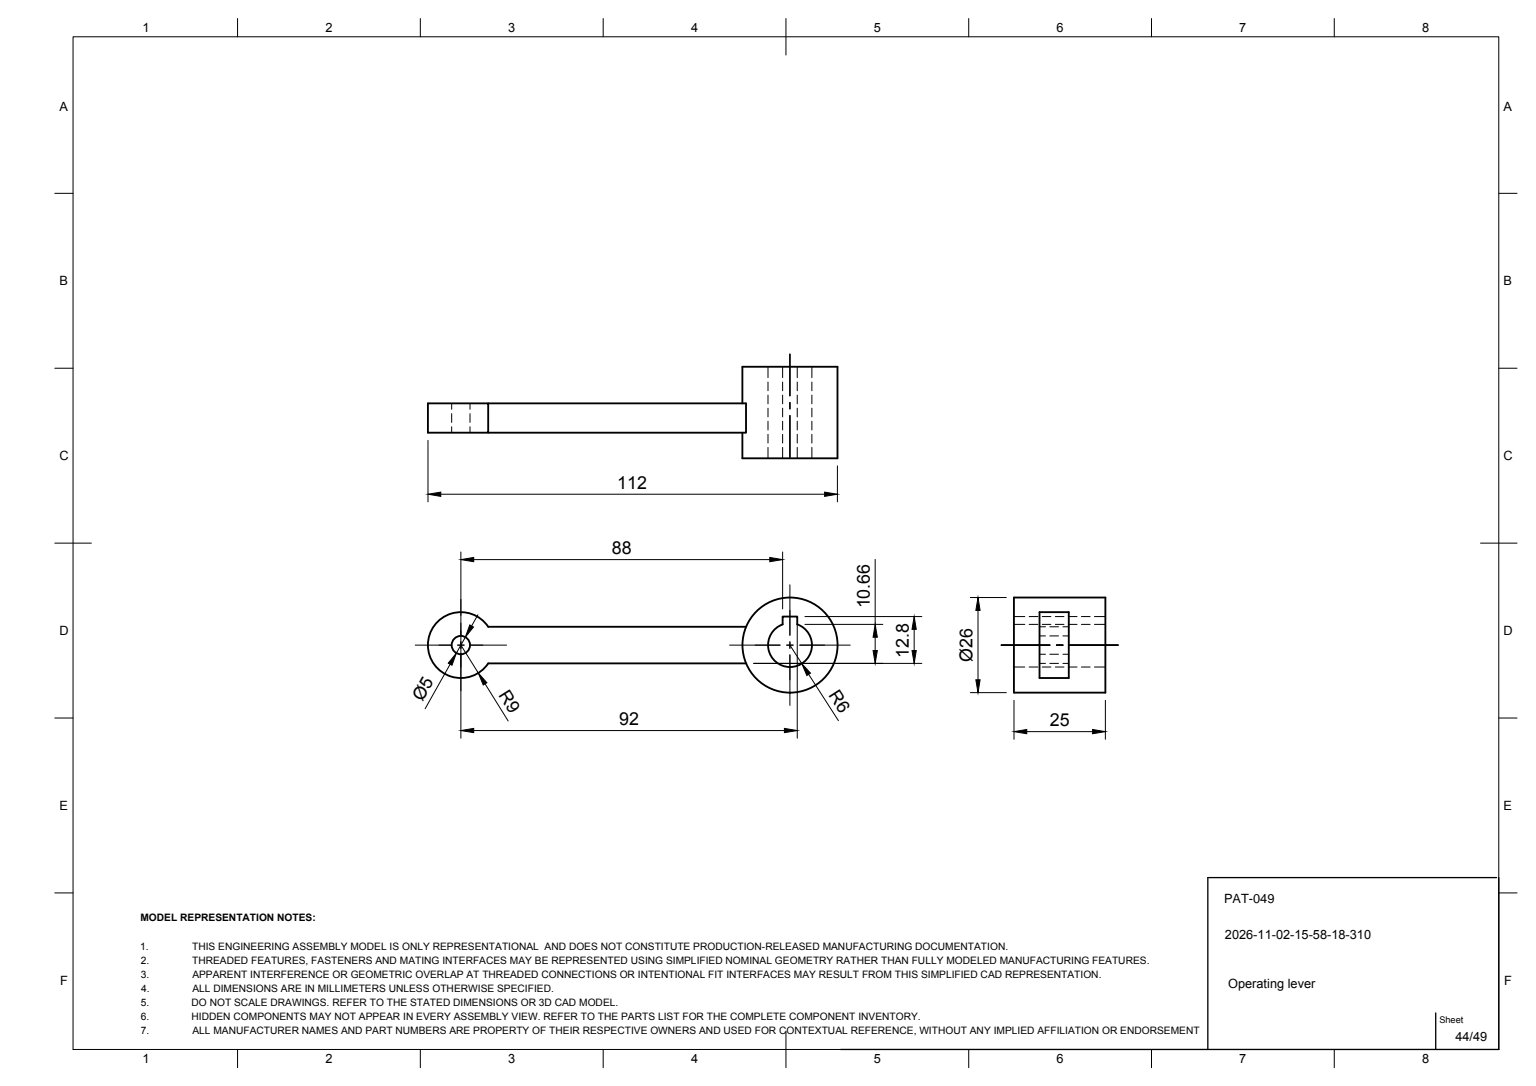
ISO-10303-21;
HEADER;
/* Generated by software containing ST-Developer
 * from STEP Tools, Inc. (www.steptools.com) 
 */

FILE_DESCRIPTION(
/* description */ ('Hand drill press frame (manual)'),
/* implementation_level */ '2;1');

FILE_NAME(
/* name */ 'Operating lever.step',
/* time_stamp */ '2026-10-28T03:25:28-07:00',
/* author */ (''),
/* organization */ (''),
/* preprocessor_version */ 'ST-DEVELOPER v20.2',
/* originating_system */ 'Autodesk Translation Framework v15.17.0.0',
/* authorisation */ '');

FILE_SCHEMA (('AUTOMOTIVE_DESIGN { 1 0 10303 214 3 1 1 }'));
ENDSEC;

DATA;
#10=MECHANICAL_DESIGN_GEOMETRIC_PRESENTATION_REPRESENTATION('',(#662),#33299);
#565=SHAPE_REPRESENTATION_RELATIONSHIP('SRR','None',#33527,#610);
#610=ADVANCED_BREP_SHAPE_REPRESENTATION('',(#713),#33289);
#662=STYLED_ITEM('',(#33800),#713);
#713=MANIFOLD_SOLID_BREP('Body1',#12681);
#867=FACE_BOUND('',#2714,.T.);
#868=FACE_BOUND('',#2719,.T.);
#869=FACE_BOUND('',#2722,.T.);
#870=FACE_BOUND('',#2724,.T.);
#871=FACE_BOUND('',#2726,.T.);
#1272=PLANE('',#14087);
#1273=PLANE('',#14088);
#1274=PLANE('',#14089);
#1275=PLANE('',#14090);
#1276=PLANE('',#14098);
#1277=PLANE('',#14099);
#1278=PLANE('',#14101);
#1279=PLANE('',#14102);
#1280=PLANE('',#14106);
#1873=FACE_OUTER_BOUND('',#2709,.T.);
#1874=FACE_OUTER_BOUND('',#2710,.T.);
#1875=FACE_OUTER_BOUND('',#2711,.T.);
#1876=FACE_OUTER_BOUND('',#2712,.T.);
#1877=FACE_OUTER_BOUND('',#2713,.T.);
#1878=FACE_OUTER_BOUND('',#2715,.T.);
#1879=FACE_OUTER_BOUND('',#2716,.T.);
#1880=FACE_OUTER_BOUND('',#2717,.T.);
#1881=FACE_OUTER_BOUND('',#2718,.T.);
#1882=FACE_OUTER_BOUND('',#2720,.T.);
#1883=FACE_OUTER_BOUND('',#2721,.T.);
#1884=FACE_OUTER_BOUND('',#2723,.T.);
#1885=FACE_OUTER_BOUND('',#2725,.T.);
#2709=EDGE_LOOP('',(#11027,#11028,#11029,#11030));
#2710=EDGE_LOOP('',(#11031,#11032,#11033,#11034));
#2711=EDGE_LOOP('',(#11035,#11036,#11037,#11038));
#2712=EDGE_LOOP('',(#11039,#11040,#11041,#11042));
#2713=EDGE_LOOP('',(#11043));
#2714=EDGE_LOOP('',(#11044,#11045,#11046,#11047));
#2715=EDGE_LOOP('',(#11048,#11049,#11050,#11051));
#2716=EDGE_LOOP('',(#11052,#11053,#11054,#11055));
#2717=EDGE_LOOP('',(#11056,#11057,#11058,#11059));
#2718=EDGE_LOOP('',(#11060,#11061,#11062,#11063));
#2719=EDGE_LOOP('',(#11064));
#2720=EDGE_LOOP('',(#11065,#11066,#11067,#11068));
#2721=EDGE_LOOP('',(#11069,#11070,#11071,#11072));
#2722=EDGE_LOOP('',(#11073));
#2723=EDGE_LOOP('',(#11074,#11075,#11076,#11077));
#2724=EDGE_LOOP('',(#11078,#11079,#11080,#11081));
#2725=EDGE_LOOP('',(#11082));
#2726=EDGE_LOOP('',(#11083,#11084,#11085,#11086));
#3840=LINE('',#21258,#5005);
#3841=LINE('',#21263,#5006);
#3842=LINE('',#21265,#5007);
#3843=LINE('',#21267,#5008);
#3844=LINE('',#21268,#5009);
#3845=LINE('',#21271,#5010);
#3846=LINE('',#21273,#5011);
#3847=LINE('',#21274,#5012);
#3848=LINE('',#21277,#5013);
#3849=LINE('',#21279,#5014);
#3850=LINE('',#21280,#5015);
#3851=LINE('',#21290,#5016);
#3852=LINE('',#21294,#5017);
#3853=LINE('',#21298,#5018);
#3854=LINE('',#21300,#5019);
#3855=LINE('',#21301,#5020);
#3856=LINE('',#21304,#5021);
#3857=LINE('',#21308,#5022);
#3858=LINE('',#21309,#5023);
#3859=LINE('',#21314,#5024);
#5005=VECTOR('',#17119,0.25);
#5006=VECTOR('',#17124,1.);
#5007=VECTOR('',#17125,1.);
#5008=VECTOR('',#17126,1.);
#5009=VECTOR('',#17127,1.);
#5010=VECTOR('',#17130,1.);
#5011=VECTOR('',#17131,1.);
#5012=VECTOR('',#17132,1.);
#5013=VECTOR('',#17135,1.);
#5014=VECTOR('',#17136,1.);
#5015=VECTOR('',#17137,1.);
#5016=VECTOR('',#17150,1.);
#5017=VECTOR('',#17153,1.);
#5018=VECTOR('',#17158,1.);
#5019=VECTOR('',#17159,1.);
#5020=VECTOR('',#17160,1.);
#5021=VECTOR('',#17163,1.);
#5022=VECTOR('',#17168,1.);
#5023=VECTOR('',#17169,1.);
#5024=VECTOR('',#17176,1.3);
#5523=CIRCLE('',#14085,0.25);
#5524=CIRCLE('',#14086,0.25);
#5525=CIRCLE('',#14091,1.3);
#5526=CIRCLE('',#14092,0.6);
#5527=CIRCLE('',#14094,0.6);
#5528=CIRCLE('',#14096,0.9);
#5529=CIRCLE('',#14097,0.9);
#5530=CIRCLE('',#14100,1.3);
#5531=CIRCLE('',#14103,1.3);
#5532=CIRCLE('',#14105,1.3);
#6489=VERTEX_POINT('',#21255);
#6490=VERTEX_POINT('',#21257);
#6491=VERTEX_POINT('',#21261);
#6492=VERTEX_POINT('',#21262);
#6493=VERTEX_POINT('',#21264);
#6494=VERTEX_POINT('',#21266);
#6495=VERTEX_POINT('',#21270);
#6496=VERTEX_POINT('',#21272);
#6497=VERTEX_POINT('',#21276);
#6498=VERTEX_POINT('',#21278);
#6499=VERTEX_POINT('',#21282);
#6500=VERTEX_POINT('',#21288);
#6501=VERTEX_POINT('',#21289);
#6502=VERTEX_POINT('',#21291);
#6503=VERTEX_POINT('',#21293);
#6504=VERTEX_POINT('',#21297);
#6505=VERTEX_POINT('',#21299);
#6506=VERTEX_POINT('',#21303);
#6507=VERTEX_POINT('',#21307);
#6508=VERTEX_POINT('',#21313);
#8042=EDGE_CURVE('',#6489,#6489,#5523,.T.);
#8043=EDGE_CURVE('',#6489,#6490,#3840,.T.);
#8044=EDGE_CURVE('',#6490,#6490,#5524,.T.);
#8045=EDGE_CURVE('',#6491,#6492,#3841,.T.);
#8046=EDGE_CURVE('',#6491,#6493,#3842,.T.);
#8047=EDGE_CURVE('',#6494,#6493,#3843,.T.);
#8048=EDGE_CURVE('',#6492,#6494,#3844,.T.);
#8049=EDGE_CURVE('',#6495,#6491,#3845,.T.);
#8050=EDGE_CURVE('',#6495,#6496,#3846,.T.);
#8051=EDGE_CURVE('',#6493,#6496,#3847,.T.);
#8052=EDGE_CURVE('',#6497,#6495,#3848,.T.);
#8053=EDGE_CURVE('',#6498,#6497,#3849,.T.);
#8054=EDGE_CURVE('',#6496,#6498,#3850,.T.);
#8055=EDGE_CURVE('',#6499,#6499,#5525,.T.);
#8056=EDGE_CURVE('',#6498,#6494,#5526,.T.);
#8057=EDGE_CURVE('',#6497,#6492,#5527,.T.);
#8058=EDGE_CURVE('',#6500,#6501,#3851,.T.);
#8059=EDGE_CURVE('',#6502,#6500,#5528,.T.);
#8060=EDGE_CURVE('',#6503,#6502,#3852,.T.);
#8061=EDGE_CURVE('',#6503,#6501,#5529,.T.);
#8062=EDGE_CURVE('',#6504,#6501,#3853,.T.);
#8063=EDGE_CURVE('',#6505,#6504,#3854,.T.);
#8064=EDGE_CURVE('',#6500,#6505,#3855,.T.);
#8065=EDGE_CURVE('',#6503,#6506,#3856,.T.);
#8066=EDGE_CURVE('',#6504,#6506,#5530,.T.);
#8067=EDGE_CURVE('',#6507,#6502,#3857,.T.);
#8068=EDGE_CURVE('',#6506,#6507,#3858,.T.);
#8069=EDGE_CURVE('',#6507,#6505,#5531,.T.);
#8070=EDGE_CURVE('',#6499,#6508,#3859,.T.);
#8071=EDGE_CURVE('',#6508,#6508,#5532,.T.);
#11027=ORIENTED_EDGE('',*,*,#8042,.F.);
#11028=ORIENTED_EDGE('',*,*,#8043,.T.);
#11029=ORIENTED_EDGE('',*,*,#8044,.F.);
#11030=ORIENTED_EDGE('',*,*,#8043,.F.);
#11031=ORIENTED_EDGE('',*,*,#8045,.F.);
#11032=ORIENTED_EDGE('',*,*,#8046,.T.);
#11033=ORIENTED_EDGE('',*,*,#8047,.F.);
#11034=ORIENTED_EDGE('',*,*,#8048,.F.);
#11035=ORIENTED_EDGE('',*,*,#8049,.F.);
#11036=ORIENTED_EDGE('',*,*,#8050,.T.);
#11037=ORIENTED_EDGE('',*,*,#8051,.F.);
#11038=ORIENTED_EDGE('',*,*,#8046,.F.);
#11039=ORIENTED_EDGE('',*,*,#8052,.F.);
#11040=ORIENTED_EDGE('',*,*,#8053,.F.);
#11041=ORIENTED_EDGE('',*,*,#8054,.F.);
#11042=ORIENTED_EDGE('',*,*,#8050,.F.);
#11043=ORIENTED_EDGE('',*,*,#8055,.T.);
#11044=ORIENTED_EDGE('',*,*,#8047,.T.);
#11045=ORIENTED_EDGE('',*,*,#8051,.T.);
#11046=ORIENTED_EDGE('',*,*,#8054,.T.);
#11047=ORIENTED_EDGE('',*,*,#8056,.T.);
#11048=ORIENTED_EDGE('',*,*,#8048,.T.);
#11049=ORIENTED_EDGE('',*,*,#8056,.F.);
#11050=ORIENTED_EDGE('',*,*,#8053,.T.);
#11051=ORIENTED_EDGE('',*,*,#8057,.T.);
#11052=ORIENTED_EDGE('',*,*,#8058,.F.);
#11053=ORIENTED_EDGE('',*,*,#8059,.F.);
#11054=ORIENTED_EDGE('',*,*,#8060,.F.);
#11055=ORIENTED_EDGE('',*,*,#8061,.T.);
#11056=ORIENTED_EDGE('',*,*,#8058,.T.);
#11057=ORIENTED_EDGE('',*,*,#8062,.F.);
#11058=ORIENTED_EDGE('',*,*,#8063,.F.);
#11059=ORIENTED_EDGE('',*,*,#8064,.F.);
#11060=ORIENTED_EDGE('',*,*,#8061,.F.);
#11061=ORIENTED_EDGE('',*,*,#8065,.T.);
#11062=ORIENTED_EDGE('',*,*,#8066,.F.);
#11063=ORIENTED_EDGE('',*,*,#8062,.T.);
#11064=ORIENTED_EDGE('',*,*,#8042,.T.);
#11065=ORIENTED_EDGE('',*,*,#8060,.T.);
#11066=ORIENTED_EDGE('',*,*,#8067,.F.);
#11067=ORIENTED_EDGE('',*,*,#8068,.F.);
#11068=ORIENTED_EDGE('',*,*,#8065,.F.);
#11069=ORIENTED_EDGE('',*,*,#8064,.T.);
#11070=ORIENTED_EDGE('',*,*,#8069,.F.);
#11071=ORIENTED_EDGE('',*,*,#8067,.T.);
#11072=ORIENTED_EDGE('',*,*,#8059,.T.);
#11073=ORIENTED_EDGE('',*,*,#8044,.T.);
#11074=ORIENTED_EDGE('',*,*,#8055,.F.);
#11075=ORIENTED_EDGE('',*,*,#8070,.T.);
#11076=ORIENTED_EDGE('',*,*,#8071,.T.);
#11077=ORIENTED_EDGE('',*,*,#8070,.F.);
#11078=ORIENTED_EDGE('',*,*,#8063,.T.);
#11079=ORIENTED_EDGE('',*,*,#8066,.T.);
#11080=ORIENTED_EDGE('',*,*,#8068,.T.);
#11081=ORIENTED_EDGE('',*,*,#8069,.T.);
#11082=ORIENTED_EDGE('',*,*,#8071,.F.);
#11083=ORIENTED_EDGE('',*,*,#8045,.T.);
#11084=ORIENTED_EDGE('',*,*,#8057,.F.);
#11085=ORIENTED_EDGE('',*,*,#8052,.T.);
#11086=ORIENTED_EDGE('',*,*,#8049,.T.);
#11908=CYLINDRICAL_SURFACE('',#14084,0.25);
#11909=CYLINDRICAL_SURFACE('',#14093,0.6);
#11910=CYLINDRICAL_SURFACE('',#14095,0.9);
#11911=CYLINDRICAL_SURFACE('',#14104,1.3);
#12482=ADVANCED_FACE('',(#1873),#11908,.F.);
#12483=ADVANCED_FACE('',(#1874),#1272,.F.);
#12484=ADVANCED_FACE('',(#1875),#1273,.F.);
#12485=ADVANCED_FACE('',(#1876),#1274,.F.);
#12486=ADVANCED_FACE('',(#1877,#867),#1275,.T.);
#12487=ADVANCED_FACE('',(#1878),#11909,.F.);
#12488=ADVANCED_FACE('',(#1879),#11910,.T.);
#12489=ADVANCED_FACE('',(#1880),#1276,.T.);
#12490=ADVANCED_FACE('',(#1881,#868),#1277,.F.);
#12491=ADVANCED_FACE('',(#1882),#1278,.T.);
#12492=ADVANCED_FACE('',(#1883,#869),#1279,.T.);
#12493=ADVANCED_FACE('',(#1884,#870),#11911,.T.);
#12494=ADVANCED_FACE('',(#1885,#871),#1280,.F.);
#12681=CLOSED_SHELL('',(#12482,#12483,#12484,#12485,#12486,#12487,#12488,
#12489,#12490,#12491,#12492,#12493,#12494));
#14083=AXIS2_PLACEMENT_3D('',#21253,#17113,#17114);
#14084=AXIS2_PLACEMENT_3D('',#21254,#17115,#17116);
#14085=AXIS2_PLACEMENT_3D('',#21256,#17117,#17118);
#14086=AXIS2_PLACEMENT_3D('',#21259,#17120,#17121);
#14087=AXIS2_PLACEMENT_3D('',#21260,#17122,#17123);
#14088=AXIS2_PLACEMENT_3D('',#21269,#17128,#17129);
#14089=AXIS2_PLACEMENT_3D('',#21275,#17133,#17134);
#14090=AXIS2_PLACEMENT_3D('',#21281,#17138,#17139);
#14091=AXIS2_PLACEMENT_3D('',#21283,#17140,#17141);
#14092=AXIS2_PLACEMENT_3D('',#21284,#17142,#17143);
#14093=AXIS2_PLACEMENT_3D('',#21285,#17144,#17145);
#14094=AXIS2_PLACEMENT_3D('',#21286,#17146,#17147);
#14095=AXIS2_PLACEMENT_3D('',#21287,#17148,#17149);
#14096=AXIS2_PLACEMENT_3D('',#21292,#17151,#17152);
#14097=AXIS2_PLACEMENT_3D('',#21295,#17154,#17155);
#14098=AXIS2_PLACEMENT_3D('',#21296,#17156,#17157);
#14099=AXIS2_PLACEMENT_3D('',#21302,#17161,#17162);
#14100=AXIS2_PLACEMENT_3D('',#21305,#17164,#17165);
#14101=AXIS2_PLACEMENT_3D('',#21306,#17166,#17167);
#14102=AXIS2_PLACEMENT_3D('',#21310,#17170,#17171);
#14103=AXIS2_PLACEMENT_3D('',#21311,#17172,#17173);
#14104=AXIS2_PLACEMENT_3D('',#21312,#17174,#17175);
#14105=AXIS2_PLACEMENT_3D('',#21315,#17177,#17178);
#14106=AXIS2_PLACEMENT_3D('',#21316,#17179,#17180);
#17113=DIRECTION('axis',(0.,0.,1.));
#17114=DIRECTION('refdir',(1.,0.,0.));
#17115=DIRECTION('center_axis',(0.,1.,0.));
#17116=DIRECTION('ref_axis',(1.,0.,0.));
#17117=DIRECTION('center_axis',(0.,1.,0.));
#17118=DIRECTION('ref_axis',(1.,0.,0.));
#17119=DIRECTION('',(0.,1.,0.));
#17120=DIRECTION('center_axis',(0.,-1.,0.));
#17121=DIRECTION('ref_axis',(1.,0.,0.));
#17122=DIRECTION('center_axis',(0.,0.,-1.));
#17123=DIRECTION('ref_axis',(-1.,0.,0.));
#17124=DIRECTION('',(-1.,0.,0.));
#17125=DIRECTION('',(0.,1.,0.));
#17126=DIRECTION('',(1.,0.,0.));
#17127=DIRECTION('',(0.,1.,0.));
#17128=DIRECTION('center_axis',(1.,0.,0.));
#17129=DIRECTION('ref_axis',(0.,0.,-1.));
#17130=DIRECTION('',(0.,0.,-1.));
#17131=DIRECTION('',(0.,1.,0.));
#17132=DIRECTION('',(0.,0.,1.));
#17133=DIRECTION('center_axis',(0.,0.,1.));
#17134=DIRECTION('ref_axis',(1.,0.,0.));
#17135=DIRECTION('',(1.,0.,0.));
#17136=DIRECTION('',(0.,-1.,0.));
#17137=DIRECTION('',(-1.,0.,0.));
#17138=DIRECTION('center_axis',(0.,1.,0.));
#17139=DIRECTION('ref_axis',(1.,0.,0.));
#17140=DIRECTION('center_axis',(0.,1.,0.));
#17141=DIRECTION('ref_axis',(1.,0.,0.));
#17142=DIRECTION('center_axis',(0.,-1.,0.));
#17143=DIRECTION('ref_axis',(1.,0.,0.));
#17144=DIRECTION('center_axis',(0.,1.,0.));
#17145=DIRECTION('ref_axis',(-1.,0.,-1.22464679914735E-16));
#17146=DIRECTION('center_axis',(0.,-1.,0.));
#17147=DIRECTION('ref_axis',(1.,0.,0.));
#17148=DIRECTION('center_axis',(0.,1.,0.));
#17149=DIRECTION('ref_axis',(6.12323399573677E-17,0.,1.));
#17150=DIRECTION('',(0.,-1.,0.));
#17151=DIRECTION('center_axis',(0.,1.,0.));
#17152=DIRECTION('ref_axis',(1.,0.,0.));
#17153=DIRECTION('',(0.,1.,0.));
#17154=DIRECTION('center_axis',(0.,1.,0.));
#17155=DIRECTION('ref_axis',(1.,0.,0.));
#17156=DIRECTION('center_axis',(1.,0.,0.));
#17157=DIRECTION('ref_axis',(0.,0.,-1.));
#17158=DIRECTION('',(0.,0.,1.));
#17159=DIRECTION('',(0.,-1.,0.));
#17160=DIRECTION('',(0.,0.,-1.));
#17161=DIRECTION('center_axis',(0.,1.,0.));
#17162=DIRECTION('ref_axis',(1.,0.,0.));
#17163=DIRECTION('',(0.,0.,-1.));
#17164=DIRECTION('center_axis',(0.,-1.,0.));
#17165=DIRECTION('ref_axis',(1.,0.,0.));
#17166=DIRECTION('center_axis',(-1.,0.,0.));
#17167=DIRECTION('ref_axis',(0.,0.,1.));
#17168=DIRECTION('',(0.,0.,1.));
#17169=DIRECTION('',(0.,1.,0.));
#17170=DIRECTION('center_axis',(0.,1.,0.));
#17171=DIRECTION('ref_axis',(0.,0.,1.));
#17172=DIRECTION('center_axis',(0.,1.,0.));
#17173=DIRECTION('ref_axis',(1.,0.,0.));
#17174=DIRECTION('center_axis',(0.,1.,0.));
#17175=DIRECTION('ref_axis',(1.,0.,0.));
#17176=DIRECTION('',(0.,-1.,0.));
#17177=DIRECTION('center_axis',(0.,1.,0.));
#17178=DIRECTION('ref_axis',(1.,0.,0.));
#17179=DIRECTION('center_axis',(0.,1.,0.));
#17180=DIRECTION('ref_axis',(1.,0.,0.));
#21253=CARTESIAN_POINT('',(0.,0.,0.));
#21254=CARTESIAN_POINT('Origin',(-3.25,5.9,29.));
#21255=CARTESIAN_POINT('',(-3.5,6.,29.));
#21256=CARTESIAN_POINT('Origin',(-3.25,6.,29.));
#21257=CARTESIAN_POINT('',(-3.5,6.8,29.));
#21258=CARTESIAN_POINT('',(-3.5,5.9,29.));
#21259=CARTESIAN_POINT('Origin',(-3.25,6.8,29.));
#21260=CARTESIAN_POINT('Origin',(-2.47,4.9,19.8));
#21261=CARTESIAN_POINT('',(-2.47,5.,19.8));
#21262=CARTESIAN_POINT('',(-2.68431457505076,5.,19.8));
#21263=CARTESIAN_POINT('',(-2.86,5.,19.8));
#21264=CARTESIAN_POINT('',(-2.47,7.5,19.8));
#21265=CARTESIAN_POINT('',(-2.47,4.9,19.8));
#21266=CARTESIAN_POINT('',(-2.68431457505076,7.5,19.8));
#21267=CARTESIAN_POINT('',(-2.86,7.5,19.8));
#21268=CARTESIAN_POINT('',(-2.68431457505076,5.,19.8));
#21269=CARTESIAN_POINT('Origin',(-2.47,4.9,20.2));
#21270=CARTESIAN_POINT('',(-2.47,5.,20.2));
#21271=CARTESIAN_POINT('',(-2.47,5.,20.1));
#21272=CARTESIAN_POINT('',(-2.47,7.5,20.2));
#21273=CARTESIAN_POINT('',(-2.47,4.9,20.2));
#21274=CARTESIAN_POINT('',(-2.47,7.5,20.1));
#21275=CARTESIAN_POINT('Origin',(-2.9,4.9,20.2));
#21276=CARTESIAN_POINT('',(-2.68431457505076,5.,20.2));
#21277=CARTESIAN_POINT('',(-3.075,5.,20.2));
#21278=CARTESIAN_POINT('',(-2.68431457505076,7.5,20.2));
#21279=CARTESIAN_POINT('',(-2.68431457505076,5.,20.2));
#21280=CARTESIAN_POINT('',(-3.075,7.5,20.2));
#21281=CARTESIAN_POINT('Origin',(-3.25,7.5,20.));
#21282=CARTESIAN_POINT('',(-4.55,7.5,20.));
#21283=CARTESIAN_POINT('Origin',(-3.25,7.5,20.));
#21284=CARTESIAN_POINT('Origin',(-3.25,7.5,20.));
#21285=CARTESIAN_POINT('Origin',(-3.25,5.,20.));
#21286=CARTESIAN_POINT('Origin',(-3.25,5.,20.));
#21287=CARTESIAN_POINT('Origin',(-3.25,6.,29.));
#21288=CARTESIAN_POINT('',(-2.75,6.8,28.2516685226452));
#21289=CARTESIAN_POINT('',(-2.75,6.,28.2516685226452));
#21290=CARTESIAN_POINT('',(-2.75,6.,28.2516685226452));
#21291=CARTESIAN_POINT('',(-3.75,6.8,28.2516685226452));
#21292=CARTESIAN_POINT('Origin',(-3.25,6.8,29.));
#21293=CARTESIAN_POINT('',(-3.75,6.,28.2516685226452));
#21294=CARTESIAN_POINT('',(-3.75,6.,28.2516685226452));
#21295=CARTESIAN_POINT('Origin',(-3.25,6.,29.));
#21296=CARTESIAN_POINT('Origin',(-2.75,6.,29.));
#21297=CARTESIAN_POINT('',(-2.75,6.,21.2));
#21298=CARTESIAN_POINT('',(-2.75,6.,20.));
#21299=CARTESIAN_POINT('',(-2.75,6.8,21.2));
#21300=CARTESIAN_POINT('',(-2.75,5.,21.2));
#21301=CARTESIAN_POINT('',(-2.75,6.8,20.));
#21302=CARTESIAN_POINT('Origin',(-3.25,6.,24.5));
#21303=CARTESIAN_POINT('',(-3.75,6.,21.2));
#21304=CARTESIAN_POINT('',(-3.75,6.,29.));
#21305=CARTESIAN_POINT('Origin',(-3.25,6.,20.));
#21306=CARTESIAN_POINT('Origin',(-3.75,6.,20.));
#21307=CARTESIAN_POINT('',(-3.75,6.8,21.2));
#21308=CARTESIAN_POINT('',(-3.75,6.8,29.));
#21309=CARTESIAN_POINT('',(-3.75,5.,21.2));
#21310=CARTESIAN_POINT('Origin',(-3.25,6.8,24.5));
#21311=CARTESIAN_POINT('Origin',(-3.25,6.8,20.));
#21312=CARTESIAN_POINT('Origin',(-3.25,5.,20.));
#21313=CARTESIAN_POINT('',(-4.55,5.,20.));
#21314=CARTESIAN_POINT('',(-4.55,5.,20.));
#21315=CARTESIAN_POINT('Origin',(-3.25,5.,20.));
#21316=CARTESIAN_POINT('Origin',(-3.25,5.,20.));
#33237=UNCERTAINTY_MEASURE_WITH_UNIT(LENGTH_MEASURE(0.001),#33300,
'DISTANCE_ACCURACY_VALUE',
'Maximum model space distance between geometric entities at asserted c
onnectivities');
#33247=UNCERTAINTY_MEASURE_WITH_UNIT(LENGTH_MEASURE(0.001),#33300,
'DISTANCE_ACCURACY_VALUE',
'Maximum model space distance between geometric entities at asserted c
onnectivities');
#33289=(
GEOMETRIC_REPRESENTATION_CONTEXT(3)
GLOBAL_UNCERTAINTY_ASSIGNED_CONTEXT((#33237))
GLOBAL_UNIT_ASSIGNED_CONTEXT((#33300,#33302,#33303))
REPRESENTATION_CONTEXT('','3D')
);
#33299=(
GEOMETRIC_REPRESENTATION_CONTEXT(3)
GLOBAL_UNCERTAINTY_ASSIGNED_CONTEXT((#33247))
GLOBAL_UNIT_ASSIGNED_CONTEXT((#33300,#33302,#33303))
REPRESENTATION_CONTEXT('','3D')
);
#33300=(
LENGTH_UNIT()
NAMED_UNIT(*)
SI_UNIT(.CENTI.,.METRE.)
);
#33302=(
NAMED_UNIT(*)
PLANE_ANGLE_UNIT()
SI_UNIT($,.RADIAN.)
);
#33303=(
NAMED_UNIT(*)
SI_UNIT($,.STERADIAN.)
SOLID_ANGLE_UNIT()
);
#33345=SHAPE_DEFINITION_REPRESENTATION(#33407,#33527);
#33407=PRODUCT_DEFINITION_SHAPE('',$,#33579);
#33527=SHAPE_REPRESENTATION('',(#14083),#33289);
#33537=PRODUCT_DEFINITION_CONTEXT('part definition',#33692,'design');
#33579=PRODUCT_DEFINITION('Operating lever','Operating lever',#33630,#33537);
#33630=PRODUCT_DEFINITION_FORMATION('',$,#33735);
#33692=APPLICATION_CONTEXT(
'Core Data for Automotive Mechanical Design Process');
#33693=PRODUCT_CONTEXT('part definition',#33692,'mechanical');
#33735=PRODUCT('Operating lever','Operating lever','Operating lever',(#33693));
#33794=COLOUR_RGB('Light Blue',0.38,0.62,0.78);
#33795=FILL_AREA_STYLE_COLOUR('',#33794);
#33796=FILL_AREA_STYLE('',(#33795));
#33797=SURFACE_STYLE_FILL_AREA(#33796);
#33798=SURFACE_SIDE_STYLE('',(#33797));
#33799=SURFACE_STYLE_USAGE(.BOTH.,#33798);
#33800=PRESENTATION_STYLE_ASSIGNMENT((#33799));
ENDSEC;
END-ISO-10303-21;
